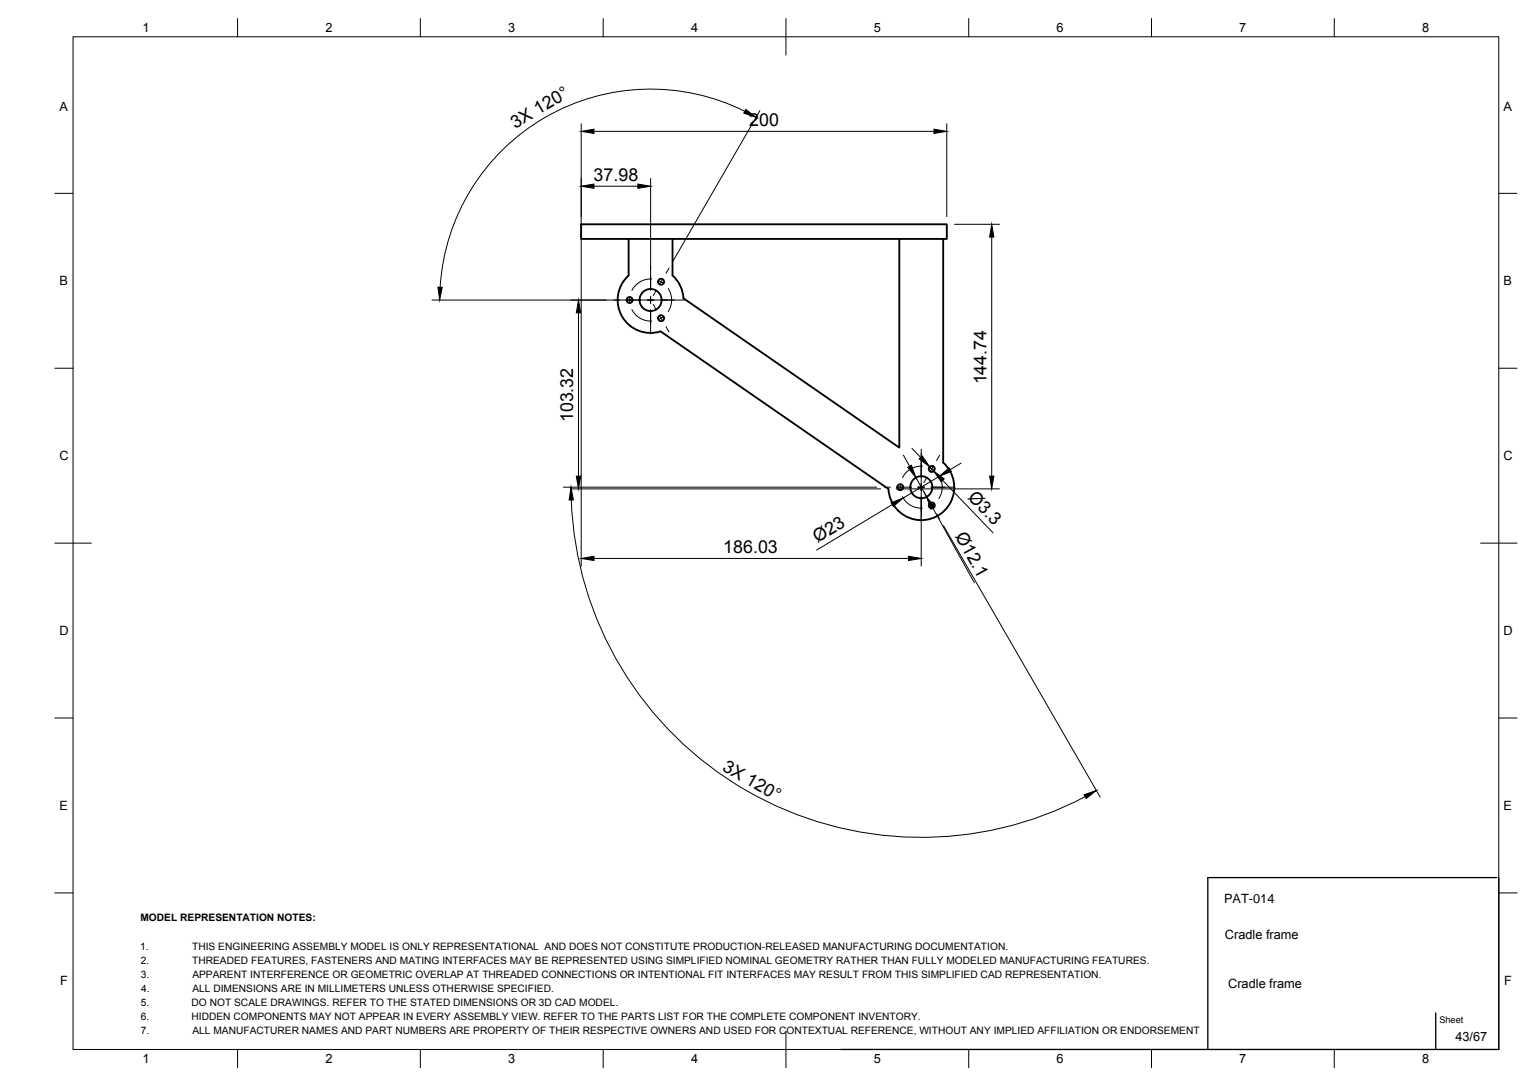
ISO-10303-21;
HEADER;
/* Generated by software containing ST-Developer
 * from STEP Tools, Inc. (www.steptools.com) 
 */

FILE_DESCRIPTION(
/* description */ ('Bin tilter linkage'),
/* implementation_level */ '2;1');

FILE_NAME(
/* name */ 'Cradle frame.step',
/* time_stamp */ '2026-10-28T03:26:24-07:00',
/* author */ (''),
/* organization */ (''),
/* preprocessor_version */ 'ST-DEVELOPER v20.2',
/* originating_system */ 'Autodesk Translation Framework v15.17.0.0',
/* authorisation */ '');

FILE_SCHEMA (('AUTOMOTIVE_DESIGN { 1 0 10303 214 3 1 1 }'));
ENDSEC;

DATA;
#10=MECHANICAL_DESIGN_GEOMETRIC_PRESENTATION_REPRESENTATION('',(#946,#947),#23728);
#727=SHAPE_REPRESENTATION_RELATIONSHIP('SRR','None',#24195,#833);
#833=ADVANCED_BREP_SHAPE_REPRESENTATION('',(#1059,#1060),#23695);
#946=STYLED_ITEM('',(#24744),#1059);
#947=STYLED_ITEM('',(#24744),#1060);
#1059=MANIFOLD_SOLID_BREP('Body1',#12477);
#1060=MANIFOLD_SOLID_BREP('Body2',#12478);
#1395=FACE_BOUND('',#3542,.T.);
#1396=FACE_BOUND('',#3543,.T.);
#1397=FACE_BOUND('',#3544,.T.);
#1398=FACE_BOUND('',#3545,.T.);
#1399=FACE_BOUND('',#3546,.T.);
#1400=FACE_BOUND('',#3547,.T.);
#1401=FACE_BOUND('',#3548,.T.);
#1402=FACE_BOUND('',#3549,.T.);
#1403=FACE_BOUND('',#3557,.T.);
#1404=FACE_BOUND('',#3558,.T.);
#1405=FACE_BOUND('',#3559,.T.);
#1406=FACE_BOUND('',#3560,.T.);
#1407=FACE_BOUND('',#3561,.T.);
#1408=FACE_BOUND('',#3562,.T.);
#1409=FACE_BOUND('',#3563,.T.);
#1410=FACE_BOUND('',#3564,.T.);
#1753=PLANE('',#14973);
#1754=PLANE('',#14974);
#1755=PLANE('',#14975);
#1756=PLANE('',#14982);
#1757=PLANE('',#14984);
#1758=PLANE('',#14985);
#1759=PLANE('',#14986);
#1760=PLANE('',#14987);
#1761=PLANE('',#14990);
#1762=PLANE('',#14991);
#1763=PLANE('',#14992);
#1764=PLANE('',#14993);
#1765=PLANE('',#14994);
#1766=PLANE('',#14995);
#1767=PLANE('',#14996);
#1768=PLANE('',#14997);
#2443=FACE_OUTER_BOUND('',#3528,.T.);
#2444=FACE_OUTER_BOUND('',#3529,.T.);
#2445=FACE_OUTER_BOUND('',#3530,.T.);
#2446=FACE_OUTER_BOUND('',#3531,.T.);
#2447=FACE_OUTER_BOUND('',#3532,.T.);
#2448=FACE_OUTER_BOUND('',#3533,.T.);
#2449=FACE_OUTER_BOUND('',#3534,.T.);
#2450=FACE_OUTER_BOUND('',#3535,.T.);
#2451=FACE_OUTER_BOUND('',#3536,.T.);
#2452=FACE_OUTER_BOUND('',#3537,.T.);
#2453=FACE_OUTER_BOUND('',#3538,.T.);
#2454=FACE_OUTER_BOUND('',#3539,.T.);
#2455=FACE_OUTER_BOUND('',#3540,.T.);
#2456=FACE_OUTER_BOUND('',#3541,.T.);
#2457=FACE_OUTER_BOUND('',#3550,.T.);
#2458=FACE_OUTER_BOUND('',#3551,.T.);
#2459=FACE_OUTER_BOUND('',#3552,.T.);
#2460=FACE_OUTER_BOUND('',#3553,.T.);
#2461=FACE_OUTER_BOUND('',#3554,.T.);
#2462=FACE_OUTER_BOUND('',#3555,.T.);
#2463=FACE_OUTER_BOUND('',#3556,.T.);
#2464=FACE_OUTER_BOUND('',#3565,.T.);
#2465=FACE_OUTER_BOUND('',#3566,.T.);
#2466=FACE_OUTER_BOUND('',#3567,.T.);
#2467=FACE_OUTER_BOUND('',#3568,.T.);
#2468=FACE_OUTER_BOUND('',#3569,.T.);
#2469=FACE_OUTER_BOUND('',#3570,.T.);
#3528=EDGE_LOOP('',(#10411,#10412,#10413,#10414));
#3529=EDGE_LOOP('',(#10415,#10416,#10417,#10418));
#3530=EDGE_LOOP('',(#10419,#10420,#10421,#10422));
#3531=EDGE_LOOP('',(#10423,#10424,#10425,#10426));
#3532=EDGE_LOOP('',(#10427,#10428,#10429,#10430));
#3533=EDGE_LOOP('',(#10431,#10432,#10433,#10434));
#3534=EDGE_LOOP('',(#10435,#10436,#10437,#10438));
#3535=EDGE_LOOP('',(#10439,#10440,#10441,#10442));
#3536=EDGE_LOOP('',(#10443,#10444,#10445,#10446));
#3537=EDGE_LOOP('',(#10447,#10448,#10449,#10450));
#3538=EDGE_LOOP('',(#10451,#10452,#10453,#10454));
#3539=EDGE_LOOP('',(#10455,#10456,#10457,#10458));
#3540=EDGE_LOOP('',(#10459,#10460,#10461,#10462));
#3541=EDGE_LOOP('',(#10463,#10464,#10465,#10466,#10467,#10468,#10469,#10470,
#10471,#10472,#10473));
#3542=EDGE_LOOP('',(#10474));
#3543=EDGE_LOOP('',(#10475));
#3544=EDGE_LOOP('',(#10476));
#3545=EDGE_LOOP('',(#10477));
#3546=EDGE_LOOP('',(#10478));
#3547=EDGE_LOOP('',(#10479));
#3548=EDGE_LOOP('',(#10480));
#3549=EDGE_LOOP('',(#10481));
#3550=EDGE_LOOP('',(#10482,#10483,#10484,#10485));
#3551=EDGE_LOOP('',(#10486,#10487,#10488,#10489));
#3552=EDGE_LOOP('',(#10490,#10491,#10492,#10493));
#3553=EDGE_LOOP('',(#10494,#10495,#10496,#10497));
#3554=EDGE_LOOP('',(#10498,#10499,#10500,#10501));
#3555=EDGE_LOOP('',(#10502,#10503,#10504,#10505));
#3556=EDGE_LOOP('',(#10506,#10507,#10508,#10509,#10510,#10511,#10512,#10513,
#10514,#10515,#10516));
#3557=EDGE_LOOP('',(#10517));
#3558=EDGE_LOOP('',(#10518));
#3559=EDGE_LOOP('',(#10519));
#3560=EDGE_LOOP('',(#10520));
#3561=EDGE_LOOP('',(#10521));
#3562=EDGE_LOOP('',(#10522));
#3563=EDGE_LOOP('',(#10523));
#3564=EDGE_LOOP('',(#10524));
#3565=EDGE_LOOP('',(#10525,#10526,#10527,#10528));
#3566=EDGE_LOOP('',(#10529,#10530,#10531,#10532));
#3567=EDGE_LOOP('',(#10533,#10534,#10535,#10536));
#3568=EDGE_LOOP('',(#10537,#10538,#10539,#10540));
#3569=EDGE_LOOP('',(#10541,#10542,#10543,#10544));
#3570=EDGE_LOOP('',(#10545,#10546,#10547,#10548));
#4269=LINE('',#22436,#4944);
#4270=LINE('',#22442,#4945);
#4271=LINE('',#22448,#4946);
#4272=LINE('',#22454,#4947);
#4273=LINE('',#22460,#4948);
#4274=LINE('',#22466,#4949);
#4275=LINE('',#22472,#4950);
#4276=LINE('',#22478,#4951);
#4277=LINE('',#22483,#4952);
#4278=LINE('',#22485,#4953);
#4279=LINE('',#22487,#4954);
#4280=LINE('',#22488,#4955);
#4281=LINE('',#22492,#4956);
#4282=LINE('',#22494,#4957);
#4283=LINE('',#22496,#4958);
#4284=LINE('',#22497,#4959);
#4285=LINE('',#22499,#4960);
#4286=LINE('',#22500,#4961);
#4287=LINE('',#22505,#4962);
#4288=LINE('',#22511,#4963);
#4289=LINE('',#22515,#4964);
#4290=LINE('',#22517,#4965);
#4291=LINE('',#22519,#4966);
#4292=LINE('',#22521,#4967);
#4293=LINE('',#22524,#4968);
#4294=LINE('',#22527,#4969);
#4295=LINE('',#22529,#4970);
#4296=LINE('',#22530,#4971);
#4297=LINE('',#22533,#4972);
#4298=LINE('',#22535,#4973);
#4299=LINE('',#22536,#4974);
#4300=LINE('',#22538,#4975);
#4301=LINE('',#22540,#4976);
#4302=LINE('',#22544,#4977);
#4303=LINE('',#22546,#4978);
#4304=LINE('',#22551,#4979);
#4305=LINE('',#22553,#4980);
#4306=LINE('',#22555,#4981);
#4307=LINE('',#22556,#4982);
#4308=LINE('',#22559,#4983);
#4309=LINE('',#22561,#4984);
#4310=LINE('',#22562,#4985);
#4311=LINE('',#22565,#4986);
#4312=LINE('',#22567,#4987);
#4313=LINE('',#22568,#4988);
#4314=LINE('',#22570,#4989);
#4315=LINE('',#22571,#4990);
#4944=VECTOR('',#18444,0.164999999999999);
#4945=VECTOR('',#18451,0.164999999999999);
#4946=VECTOR('',#18458,0.164999999999999);
#4947=VECTOR('',#18465,0.605);
#4948=VECTOR('',#18472,0.164999999999999);
#4949=VECTOR('',#18479,0.164999999999999);
#4950=VECTOR('',#18486,0.164999999999999);
#4951=VECTOR('',#18493,0.605);
#4952=VECTOR('',#18498,1.);
#4953=VECTOR('',#18499,1.);
#4954=VECTOR('',#18500,1.);
#4955=VECTOR('',#18501,1.);
#4956=VECTOR('',#18504,1.);
#4957=VECTOR('',#18505,1.);
#4958=VECTOR('',#18506,1.);
#4959=VECTOR('',#18507,1.);
#4960=VECTOR('',#18510,1.);
#4961=VECTOR('',#18511,1.);
#4962=VECTOR('',#18516,1.);
#4963=VECTOR('',#18523,1.);
#4964=VECTOR('',#18528,1.);
#4965=VECTOR('',#18529,1.);
#4966=VECTOR('',#18530,1.);
#4967=VECTOR('',#18531,1.);
#4968=VECTOR('',#18534,1.);
#4969=VECTOR('',#18537,1.);
#4970=VECTOR('',#18538,1.);
#4971=VECTOR('',#18539,1.);
#4972=VECTOR('',#18542,1.);
#4973=VECTOR('',#18543,1.);
#4974=VECTOR('',#18544,1.);
#4975=VECTOR('',#18547,1.);
#4976=VECTOR('',#18550,1.);
#4977=VECTOR('',#18555,1.);
#4978=VECTOR('',#18558,1.);
#4979=VECTOR('',#18563,1.);
#4980=VECTOR('',#18564,1.);
#4981=VECTOR('',#18565,1.);
#4982=VECTOR('',#18566,1.);
#4983=VECTOR('',#18569,1.);
#4984=VECTOR('',#18570,1.);
#4985=VECTOR('',#18571,1.);
#4986=VECTOR('',#18574,1.);
#4987=VECTOR('',#18575,1.);
#4988=VECTOR('',#18576,1.);
#4989=VECTOR('',#18579,1.);
#4990=VECTOR('',#18580,1.);
#5784=CIRCLE('',#14950,0.164999999999999);
#5785=CIRCLE('',#14951,0.164999999999999);
#5786=CIRCLE('',#14953,0.164999999999999);
#5787=CIRCLE('',#14954,0.164999999999999);
#5788=CIRCLE('',#14956,0.164999999999999);
#5789=CIRCLE('',#14957,0.164999999999999);
#5790=CIRCLE('',#14959,0.605);
#5791=CIRCLE('',#14960,0.605);
#5792=CIRCLE('',#14962,0.164999999999999);
#5793=CIRCLE('',#14963,0.164999999999999);
#5794=CIRCLE('',#14965,0.164999999999999);
#5795=CIRCLE('',#14966,0.164999999999999);
#5796=CIRCLE('',#14968,0.164999999999999);
#5797=CIRCLE('',#14969,0.164999999999999);
#5798=CIRCLE('',#14971,0.605);
#5799=CIRCLE('',#14972,0.605);
#5800=CIRCLE('',#14977,1.8);
#5801=CIRCLE('',#14978,1.8);
#5802=CIRCLE('',#14980,1.8);
#5803=CIRCLE('',#14981,1.8);
#5804=CIRCLE('',#14983,1.8);
#5805=CIRCLE('',#14989,1.8);
#6643=VERTEX_POINT('',#22433);
#6644=VERTEX_POINT('',#22435);
#6645=VERTEX_POINT('',#22439);
#6646=VERTEX_POINT('',#22441);
#6647=VERTEX_POINT('',#22445);
#6648=VERTEX_POINT('',#22447);
#6649=VERTEX_POINT('',#22451);
#6650=VERTEX_POINT('',#22453);
#6651=VERTEX_POINT('',#22457);
#6652=VERTEX_POINT('',#22459);
#6653=VERTEX_POINT('',#22463);
#6654=VERTEX_POINT('',#22465);
#6655=VERTEX_POINT('',#22469);
#6656=VERTEX_POINT('',#22471);
#6657=VERTEX_POINT('',#22475);
#6658=VERTEX_POINT('',#22477);
#6659=VERTEX_POINT('',#22481);
#6660=VERTEX_POINT('',#22482);
#6661=VERTEX_POINT('',#22484);
#6662=VERTEX_POINT('',#22486);
#6663=VERTEX_POINT('',#22490);
#6664=VERTEX_POINT('',#22491);
#6665=VERTEX_POINT('',#22493);
#6666=VERTEX_POINT('',#22495);
#6667=VERTEX_POINT('',#22502);
#6668=VERTEX_POINT('',#22504);
#6669=VERTEX_POINT('',#22508);
#6670=VERTEX_POINT('',#22510);
#6671=VERTEX_POINT('',#22514);
#6672=VERTEX_POINT('',#22516);
#6673=VERTEX_POINT('',#22518);
#6674=VERTEX_POINT('',#22520);
#6675=VERTEX_POINT('',#22522);
#6676=VERTEX_POINT('',#22526);
#6677=VERTEX_POINT('',#22528);
#6678=VERTEX_POINT('',#22532);
#6679=VERTEX_POINT('',#22534);
#6680=VERTEX_POINT('',#22542);
#6681=VERTEX_POINT('',#22549);
#6682=VERTEX_POINT('',#22550);
#6683=VERTEX_POINT('',#22552);
#6684=VERTEX_POINT('',#22554);
#6685=VERTEX_POINT('',#22558);
#6686=VERTEX_POINT('',#22560);
#6687=VERTEX_POINT('',#22564);
#6688=VERTEX_POINT('',#22566);
#7945=EDGE_CURVE('',#6643,#6643,#5784,.T.);
#7946=EDGE_CURVE('',#6643,#6644,#4269,.T.);
#7947=EDGE_CURVE('',#6644,#6644,#5785,.T.);
#7948=EDGE_CURVE('',#6645,#6645,#5786,.T.);
#7949=EDGE_CURVE('',#6645,#6646,#4270,.T.);
#7950=EDGE_CURVE('',#6646,#6646,#5787,.T.);
#7951=EDGE_CURVE('',#6647,#6647,#5788,.T.);
#7952=EDGE_CURVE('',#6647,#6648,#4271,.T.);
#7953=EDGE_CURVE('',#6648,#6648,#5789,.T.);
#7954=EDGE_CURVE('',#6649,#6649,#5790,.T.);
#7955=EDGE_CURVE('',#6649,#6650,#4272,.T.);
#7956=EDGE_CURVE('',#6650,#6650,#5791,.T.);
#7957=EDGE_CURVE('',#6651,#6651,#5792,.T.);
#7958=EDGE_CURVE('',#6651,#6652,#4273,.T.);
#7959=EDGE_CURVE('',#6652,#6652,#5793,.T.);
#7960=EDGE_CURVE('',#6653,#6653,#5794,.T.);
#7961=EDGE_CURVE('',#6653,#6654,#4274,.T.);
#7962=EDGE_CURVE('',#6654,#6654,#5795,.T.);
#7963=EDGE_CURVE('',#6655,#6655,#5796,.T.);
#7964=EDGE_CURVE('',#6655,#6656,#4275,.T.);
#7965=EDGE_CURVE('',#6656,#6656,#5797,.T.);
#7966=EDGE_CURVE('',#6657,#6657,#5798,.T.);
#7967=EDGE_CURVE('',#6657,#6658,#4276,.T.);
#7968=EDGE_CURVE('',#6658,#6658,#5799,.T.);
#7969=EDGE_CURVE('',#6659,#6660,#4277,.T.);
#7970=EDGE_CURVE('',#6661,#6659,#4278,.T.);
#7971=EDGE_CURVE('',#6661,#6662,#4279,.T.);
#7972=EDGE_CURVE('',#6660,#6662,#4280,.T.);
#7973=EDGE_CURVE('',#6663,#6664,#4281,.T.);
#7974=EDGE_CURVE('',#6665,#6663,#4282,.T.);
#7975=EDGE_CURVE('',#6666,#6665,#4283,.T.);
#7976=EDGE_CURVE('',#6664,#6666,#4284,.T.);
#7977=EDGE_CURVE('',#6666,#6661,#4285,.T.);
#7978=EDGE_CURVE('',#6662,#6665,#4286,.T.);
#7979=EDGE_CURVE('',#6667,#6660,#5800,.T.);
#7980=EDGE_CURVE('',#6668,#6667,#4287,.T.);
#7981=EDGE_CURVE('',#6668,#6659,#5801,.T.);
#7982=EDGE_CURVE('',#6664,#6669,#5802,.T.);
#7983=EDGE_CURVE('',#6670,#6669,#4288,.T.);
#7984=EDGE_CURVE('',#6663,#6670,#5803,.T.);
#7985=EDGE_CURVE('',#6671,#6668,#4289,.T.);
#7986=EDGE_CURVE('',#6671,#6672,#4290,.T.);
#7987=EDGE_CURVE('',#6672,#6673,#4291,.T.);
#7988=EDGE_CURVE('',#6673,#6674,#4292,.T.);
#7989=EDGE_CURVE('',#6675,#6674,#5804,.T.);
#7990=EDGE_CURVE('',#6669,#6675,#4293,.T.);
#7991=EDGE_CURVE('',#6674,#6676,#4294,.T.);
#7992=EDGE_CURVE('',#6673,#6677,#4295,.T.);
#7993=EDGE_CURVE('',#6676,#6677,#4296,.T.);
#7994=EDGE_CURVE('',#6678,#6671,#4297,.T.);
#7995=EDGE_CURVE('',#6679,#6678,#4298,.T.);
#7996=EDGE_CURVE('',#6672,#6679,#4299,.T.);
#7997=EDGE_CURVE('',#6677,#6679,#4300,.T.);
#7998=EDGE_CURVE('',#6678,#6667,#4301,.T.);
#7999=EDGE_CURVE('',#6680,#6676,#5805,.T.);
#8000=EDGE_CURVE('',#6675,#6680,#4302,.T.);
#8001=EDGE_CURVE('',#6670,#6680,#4303,.T.);
#8002=EDGE_CURVE('',#6681,#6682,#4304,.T.);
#8003=EDGE_CURVE('',#6682,#6683,#4305,.T.);
#8004=EDGE_CURVE('',#6684,#6683,#4306,.T.);
#8005=EDGE_CURVE('',#6681,#6684,#4307,.T.);
#8006=EDGE_CURVE('',#6685,#6681,#4308,.T.);
#8007=EDGE_CURVE('',#6686,#6684,#4309,.T.);
#8008=EDGE_CURVE('',#6685,#6686,#4310,.T.);
#8009=EDGE_CURVE('',#6687,#6685,#4311,.T.);
#8010=EDGE_CURVE('',#6688,#6686,#4312,.T.);
#8011=EDGE_CURVE('',#6687,#6688,#4313,.T.);
#8012=EDGE_CURVE('',#6682,#6687,#4314,.T.);
#8013=EDGE_CURVE('',#6683,#6688,#4315,.T.);
#10411=ORIENTED_EDGE('',*,*,#7945,.F.);
#10412=ORIENTED_EDGE('',*,*,#7946,.T.);
#10413=ORIENTED_EDGE('',*,*,#7947,.F.);
#10414=ORIENTED_EDGE('',*,*,#7946,.F.);
#10415=ORIENTED_EDGE('',*,*,#7948,.F.);
#10416=ORIENTED_EDGE('',*,*,#7949,.T.);
#10417=ORIENTED_EDGE('',*,*,#7950,.F.);
#10418=ORIENTED_EDGE('',*,*,#7949,.F.);
#10419=ORIENTED_EDGE('',*,*,#7951,.F.);
#10420=ORIENTED_EDGE('',*,*,#7952,.T.);
#10421=ORIENTED_EDGE('',*,*,#7953,.F.);
#10422=ORIENTED_EDGE('',*,*,#7952,.F.);
#10423=ORIENTED_EDGE('',*,*,#7954,.F.);
#10424=ORIENTED_EDGE('',*,*,#7955,.T.);
#10425=ORIENTED_EDGE('',*,*,#7956,.F.);
#10426=ORIENTED_EDGE('',*,*,#7955,.F.);
#10427=ORIENTED_EDGE('',*,*,#7957,.F.);
#10428=ORIENTED_EDGE('',*,*,#7958,.T.);
#10429=ORIENTED_EDGE('',*,*,#7959,.F.);
#10430=ORIENTED_EDGE('',*,*,#7958,.F.);
#10431=ORIENTED_EDGE('',*,*,#7960,.F.);
#10432=ORIENTED_EDGE('',*,*,#7961,.T.);
#10433=ORIENTED_EDGE('',*,*,#7962,.F.);
#10434=ORIENTED_EDGE('',*,*,#7961,.F.);
#10435=ORIENTED_EDGE('',*,*,#7963,.F.);
#10436=ORIENTED_EDGE('',*,*,#7964,.T.);
#10437=ORIENTED_EDGE('',*,*,#7965,.F.);
#10438=ORIENTED_EDGE('',*,*,#7964,.F.);
#10439=ORIENTED_EDGE('',*,*,#7966,.F.);
#10440=ORIENTED_EDGE('',*,*,#7967,.T.);
#10441=ORIENTED_EDGE('',*,*,#7968,.F.);
#10442=ORIENTED_EDGE('',*,*,#7967,.F.);
#10443=ORIENTED_EDGE('',*,*,#7969,.F.);
#10444=ORIENTED_EDGE('',*,*,#7970,.F.);
#10445=ORIENTED_EDGE('',*,*,#7971,.T.);
#10446=ORIENTED_EDGE('',*,*,#7972,.F.);
#10447=ORIENTED_EDGE('',*,*,#7973,.F.);
#10448=ORIENTED_EDGE('',*,*,#7974,.F.);
#10449=ORIENTED_EDGE('',*,*,#7975,.F.);
#10450=ORIENTED_EDGE('',*,*,#7976,.F.);
#10451=ORIENTED_EDGE('',*,*,#7977,.F.);
#10452=ORIENTED_EDGE('',*,*,#7975,.T.);
#10453=ORIENTED_EDGE('',*,*,#7978,.F.);
#10454=ORIENTED_EDGE('',*,*,#7971,.F.);
#10455=ORIENTED_EDGE('',*,*,#7969,.T.);
#10456=ORIENTED_EDGE('',*,*,#7979,.F.);
#10457=ORIENTED_EDGE('',*,*,#7980,.F.);
#10458=ORIENTED_EDGE('',*,*,#7981,.T.);
#10459=ORIENTED_EDGE('',*,*,#7973,.T.);
#10460=ORIENTED_EDGE('',*,*,#7982,.T.);
#10461=ORIENTED_EDGE('',*,*,#7983,.F.);
#10462=ORIENTED_EDGE('',*,*,#7984,.F.);
#10463=ORIENTED_EDGE('',*,*,#7981,.F.);
#10464=ORIENTED_EDGE('',*,*,#7985,.F.);
#10465=ORIENTED_EDGE('',*,*,#7986,.T.);
#10466=ORIENTED_EDGE('',*,*,#7987,.T.);
#10467=ORIENTED_EDGE('',*,*,#7988,.T.);
#10468=ORIENTED_EDGE('',*,*,#7989,.F.);
#10469=ORIENTED_EDGE('',*,*,#7990,.F.);
#10470=ORIENTED_EDGE('',*,*,#7982,.F.);
#10471=ORIENTED_EDGE('',*,*,#7976,.T.);
#10472=ORIENTED_EDGE('',*,*,#7977,.T.);
#10473=ORIENTED_EDGE('',*,*,#7970,.T.);
#10474=ORIENTED_EDGE('',*,*,#7966,.T.);
#10475=ORIENTED_EDGE('',*,*,#7963,.T.);
#10476=ORIENTED_EDGE('',*,*,#7960,.T.);
#10477=ORIENTED_EDGE('',*,*,#7957,.T.);
#10478=ORIENTED_EDGE('',*,*,#7954,.T.);
#10479=ORIENTED_EDGE('',*,*,#7951,.T.);
#10480=ORIENTED_EDGE('',*,*,#7948,.T.);
#10481=ORIENTED_EDGE('',*,*,#7945,.T.);
#10482=ORIENTED_EDGE('',*,*,#7991,.F.);
#10483=ORIENTED_EDGE('',*,*,#7988,.F.);
#10484=ORIENTED_EDGE('',*,*,#7992,.T.);
#10485=ORIENTED_EDGE('',*,*,#7993,.F.);
#10486=ORIENTED_EDGE('',*,*,#7994,.F.);
#10487=ORIENTED_EDGE('',*,*,#7995,.F.);
#10488=ORIENTED_EDGE('',*,*,#7996,.F.);
#10489=ORIENTED_EDGE('',*,*,#7986,.F.);
#10490=ORIENTED_EDGE('',*,*,#7987,.F.);
#10491=ORIENTED_EDGE('',*,*,#7996,.T.);
#10492=ORIENTED_EDGE('',*,*,#7997,.F.);
#10493=ORIENTED_EDGE('',*,*,#7992,.F.);
#10494=ORIENTED_EDGE('',*,*,#7994,.T.);
#10495=ORIENTED_EDGE('',*,*,#7985,.T.);
#10496=ORIENTED_EDGE('',*,*,#7980,.T.);
#10497=ORIENTED_EDGE('',*,*,#7998,.F.);
#10498=ORIENTED_EDGE('',*,*,#7991,.T.);
#10499=ORIENTED_EDGE('',*,*,#7999,.F.);
#10500=ORIENTED_EDGE('',*,*,#8000,.F.);
#10501=ORIENTED_EDGE('',*,*,#7989,.T.);
#10502=ORIENTED_EDGE('',*,*,#7983,.T.);
#10503=ORIENTED_EDGE('',*,*,#7990,.T.);
#10504=ORIENTED_EDGE('',*,*,#8000,.T.);
#10505=ORIENTED_EDGE('',*,*,#8001,.F.);
#10506=ORIENTED_EDGE('',*,*,#7984,.T.);
#10507=ORIENTED_EDGE('',*,*,#8001,.T.);
#10508=ORIENTED_EDGE('',*,*,#7999,.T.);
#10509=ORIENTED_EDGE('',*,*,#7993,.T.);
#10510=ORIENTED_EDGE('',*,*,#7997,.T.);
#10511=ORIENTED_EDGE('',*,*,#7995,.T.);
#10512=ORIENTED_EDGE('',*,*,#7998,.T.);
#10513=ORIENTED_EDGE('',*,*,#7979,.T.);
#10514=ORIENTED_EDGE('',*,*,#7972,.T.);
#10515=ORIENTED_EDGE('',*,*,#7978,.T.);
#10516=ORIENTED_EDGE('',*,*,#7974,.T.);
#10517=ORIENTED_EDGE('',*,*,#7968,.T.);
#10518=ORIENTED_EDGE('',*,*,#7965,.T.);
#10519=ORIENTED_EDGE('',*,*,#7962,.T.);
#10520=ORIENTED_EDGE('',*,*,#7959,.T.);
#10521=ORIENTED_EDGE('',*,*,#7956,.T.);
#10522=ORIENTED_EDGE('',*,*,#7953,.T.);
#10523=ORIENTED_EDGE('',*,*,#7950,.T.);
#10524=ORIENTED_EDGE('',*,*,#7947,.T.);
#10525=ORIENTED_EDGE('',*,*,#8002,.T.);
#10526=ORIENTED_EDGE('',*,*,#8003,.T.);
#10527=ORIENTED_EDGE('',*,*,#8004,.F.);
#10528=ORIENTED_EDGE('',*,*,#8005,.F.);
#10529=ORIENTED_EDGE('',*,*,#8006,.T.);
#10530=ORIENTED_EDGE('',*,*,#8005,.T.);
#10531=ORIENTED_EDGE('',*,*,#8007,.F.);
#10532=ORIENTED_EDGE('',*,*,#8008,.F.);
#10533=ORIENTED_EDGE('',*,*,#8009,.T.);
#10534=ORIENTED_EDGE('',*,*,#8008,.T.);
#10535=ORIENTED_EDGE('',*,*,#8010,.F.);
#10536=ORIENTED_EDGE('',*,*,#8011,.F.);
#10537=ORIENTED_EDGE('',*,*,#8012,.T.);
#10538=ORIENTED_EDGE('',*,*,#8011,.T.);
#10539=ORIENTED_EDGE('',*,*,#8013,.F.);
#10540=ORIENTED_EDGE('',*,*,#8003,.F.);
#10541=ORIENTED_EDGE('',*,*,#8013,.T.);
#10542=ORIENTED_EDGE('',*,*,#8010,.T.);
#10543=ORIENTED_EDGE('',*,*,#8007,.T.);
#10544=ORIENTED_EDGE('',*,*,#8004,.T.);
#10545=ORIENTED_EDGE('',*,*,#8012,.F.);
#10546=ORIENTED_EDGE('',*,*,#8002,.F.);
#10547=ORIENTED_EDGE('',*,*,#8006,.F.);
#10548=ORIENTED_EDGE('',*,*,#8009,.F.);
#11535=CYLINDRICAL_SURFACE('',#14949,0.164999999999999);
#11536=CYLINDRICAL_SURFACE('',#14952,0.164999999999999);
#11537=CYLINDRICAL_SURFACE('',#14955,0.164999999999999);
#11538=CYLINDRICAL_SURFACE('',#14958,0.605);
#11539=CYLINDRICAL_SURFACE('',#14961,0.164999999999999);
#11540=CYLINDRICAL_SURFACE('',#14964,0.164999999999999);
#11541=CYLINDRICAL_SURFACE('',#14967,0.164999999999999);
#11542=CYLINDRICAL_SURFACE('',#14970,0.605);
#11543=CYLINDRICAL_SURFACE('',#14976,1.8);
#11544=CYLINDRICAL_SURFACE('',#14979,1.8);
#11545=CYLINDRICAL_SURFACE('',#14988,1.8);
#12168=ADVANCED_FACE('',(#2443),#11535,.F.);
#12169=ADVANCED_FACE('',(#2444),#11536,.F.);
#12170=ADVANCED_FACE('',(#2445),#11537,.F.);
#12171=ADVANCED_FACE('',(#2446),#11538,.F.);
#12172=ADVANCED_FACE('',(#2447),#11539,.F.);
#12173=ADVANCED_FACE('',(#2448),#11540,.F.);
#12174=ADVANCED_FACE('',(#2449),#11541,.F.);
#12175=ADVANCED_FACE('',(#2450),#11542,.F.);
#12176=ADVANCED_FACE('',(#2451),#1753,.T.);
#12177=ADVANCED_FACE('',(#2452),#1754,.T.);
#12178=ADVANCED_FACE('',(#2453),#1755,.T.);
#12179=ADVANCED_FACE('',(#2454),#11543,.T.);
#12180=ADVANCED_FACE('',(#2455),#11544,.T.);
#12181=ADVANCED_FACE('',(#2456,#1395,#1396,#1397,#1398,#1399,#1400,#1401,
#1402),#1756,.F.);
#12182=ADVANCED_FACE('',(#2457),#1757,.T.);
#12183=ADVANCED_FACE('',(#2458),#1758,.T.);
#12184=ADVANCED_FACE('',(#2459),#1759,.T.);
#12185=ADVANCED_FACE('',(#2460),#1760,.T.);
#12186=ADVANCED_FACE('',(#2461),#11545,.T.);
#12187=ADVANCED_FACE('',(#2462),#1761,.T.);
#12188=ADVANCED_FACE('',(#2463,#1403,#1404,#1405,#1406,#1407,#1408,#1409,
#1410),#1762,.T.);
#12189=ADVANCED_FACE('',(#2464),#1763,.T.);
#12190=ADVANCED_FACE('',(#2465),#1764,.T.);
#12191=ADVANCED_FACE('',(#2466),#1765,.T.);
#12192=ADVANCED_FACE('',(#2467),#1766,.T.);
#12193=ADVANCED_FACE('',(#2468),#1767,.T.);
#12194=ADVANCED_FACE('',(#2469),#1768,.F.);
#12477=CLOSED_SHELL('',(#12168,#12169,#12170,#12171,#12172,#12173,#12174,
#12175,#12176,#12177,#12178,#12179,#12180,#12181,#12182,#12183,#12184,#12185,
#12186,#12187,#12188));
#12478=CLOSED_SHELL('',(#12189,#12190,#12191,#12192,#12193,#12194));
#14948=AXIS2_PLACEMENT_3D('',#22431,#18438,#18439);
#14949=AXIS2_PLACEMENT_3D('',#22432,#18440,#18441);
#14950=AXIS2_PLACEMENT_3D('',#22434,#18442,#18443);
#14951=AXIS2_PLACEMENT_3D('',#22437,#18445,#18446);
#14952=AXIS2_PLACEMENT_3D('',#22438,#18447,#18448);
#14953=AXIS2_PLACEMENT_3D('',#22440,#18449,#18450);
#14954=AXIS2_PLACEMENT_3D('',#22443,#18452,#18453);
#14955=AXIS2_PLACEMENT_3D('',#22444,#18454,#18455);
#14956=AXIS2_PLACEMENT_3D('',#22446,#18456,#18457);
#14957=AXIS2_PLACEMENT_3D('',#22449,#18459,#18460);
#14958=AXIS2_PLACEMENT_3D('',#22450,#18461,#18462);
#14959=AXIS2_PLACEMENT_3D('',#22452,#18463,#18464);
#14960=AXIS2_PLACEMENT_3D('',#22455,#18466,#18467);
#14961=AXIS2_PLACEMENT_3D('',#22456,#18468,#18469);
#14962=AXIS2_PLACEMENT_3D('',#22458,#18470,#18471);
#14963=AXIS2_PLACEMENT_3D('',#22461,#18473,#18474);
#14964=AXIS2_PLACEMENT_3D('',#22462,#18475,#18476);
#14965=AXIS2_PLACEMENT_3D('',#22464,#18477,#18478);
#14966=AXIS2_PLACEMENT_3D('',#22467,#18480,#18481);
#14967=AXIS2_PLACEMENT_3D('',#22468,#18482,#18483);
#14968=AXIS2_PLACEMENT_3D('',#22470,#18484,#18485);
#14969=AXIS2_PLACEMENT_3D('',#22473,#18487,#18488);
#14970=AXIS2_PLACEMENT_3D('',#22474,#18489,#18490);
#14971=AXIS2_PLACEMENT_3D('',#22476,#18491,#18492);
#14972=AXIS2_PLACEMENT_3D('',#22479,#18494,#18495);
#14973=AXIS2_PLACEMENT_3D('',#22480,#18496,#18497);
#14974=AXIS2_PLACEMENT_3D('',#22489,#18502,#18503);
#14975=AXIS2_PLACEMENT_3D('',#22498,#18508,#18509);
#14976=AXIS2_PLACEMENT_3D('',#22501,#18512,#18513);
#14977=AXIS2_PLACEMENT_3D('',#22503,#18514,#18515);
#14978=AXIS2_PLACEMENT_3D('',#22506,#18517,#18518);
#14979=AXIS2_PLACEMENT_3D('',#22507,#18519,#18520);
#14980=AXIS2_PLACEMENT_3D('',#22509,#18521,#18522);
#14981=AXIS2_PLACEMENT_3D('',#22512,#18524,#18525);
#14982=AXIS2_PLACEMENT_3D('',#22513,#18526,#18527);
#14983=AXIS2_PLACEMENT_3D('',#22523,#18532,#18533);
#14984=AXIS2_PLACEMENT_3D('',#22525,#18535,#18536);
#14985=AXIS2_PLACEMENT_3D('',#22531,#18540,#18541);
#14986=AXIS2_PLACEMENT_3D('',#22537,#18545,#18546);
#14987=AXIS2_PLACEMENT_3D('',#22539,#18548,#18549);
#14988=AXIS2_PLACEMENT_3D('',#22541,#18551,#18552);
#14989=AXIS2_PLACEMENT_3D('',#22543,#18553,#18554);
#14990=AXIS2_PLACEMENT_3D('',#22545,#18556,#18557);
#14991=AXIS2_PLACEMENT_3D('',#22547,#18559,#18560);
#14992=AXIS2_PLACEMENT_3D('',#22548,#18561,#18562);
#14993=AXIS2_PLACEMENT_3D('',#22557,#18567,#18568);
#14994=AXIS2_PLACEMENT_3D('',#22563,#18572,#18573);
#14995=AXIS2_PLACEMENT_3D('',#22569,#18577,#18578);
#14996=AXIS2_PLACEMENT_3D('',#22572,#18581,#18582);
#14997=AXIS2_PLACEMENT_3D('',#22573,#18583,#18584);
#18438=DIRECTION('axis',(0.,0.,1.));
#18439=DIRECTION('refdir',(1.,0.,0.));
#18440=DIRECTION('center_axis',(0.,1.,0.));
#18441=DIRECTION('ref_axis',(1.,0.,0.));
#18442=DIRECTION('center_axis',(0.,1.,0.));
#18443=DIRECTION('ref_axis',(1.,0.,0.));
#18444=DIRECTION('',(0.,1.,0.));
#18445=DIRECTION('center_axis',(0.,-1.,0.));
#18446=DIRECTION('ref_axis',(1.,0.,0.));
#18447=DIRECTION('center_axis',(0.,1.,0.));
#18448=DIRECTION('ref_axis',(1.,0.,0.));
#18449=DIRECTION('center_axis',(0.,1.,0.));
#18450=DIRECTION('ref_axis',(1.,0.,0.));
#18451=DIRECTION('',(0.,1.,0.));
#18452=DIRECTION('center_axis',(0.,-1.,0.));
#18453=DIRECTION('ref_axis',(1.,0.,0.));
#18454=DIRECTION('center_axis',(0.,1.,0.));
#18455=DIRECTION('ref_axis',(1.,0.,0.));
#18456=DIRECTION('center_axis',(0.,1.,0.));
#18457=DIRECTION('ref_axis',(1.,0.,0.));
#18458=DIRECTION('',(0.,1.,0.));
#18459=DIRECTION('center_axis',(0.,-1.,0.));
#18460=DIRECTION('ref_axis',(1.,0.,0.));
#18461=DIRECTION('center_axis',(0.,1.,0.));
#18462=DIRECTION('ref_axis',(1.,0.,0.));
#18463=DIRECTION('center_axis',(0.,1.,0.));
#18464=DIRECTION('ref_axis',(1.,0.,0.));
#18465=DIRECTION('',(0.,1.,0.));
#18466=DIRECTION('center_axis',(0.,-1.,0.));
#18467=DIRECTION('ref_axis',(1.,0.,0.));
#18468=DIRECTION('center_axis',(0.,1.,0.));
#18469=DIRECTION('ref_axis',(1.,0.,0.));
#18470=DIRECTION('center_axis',(0.,1.,0.));
#18471=DIRECTION('ref_axis',(1.,0.,0.));
#18472=DIRECTION('',(0.,1.,0.));
#18473=DIRECTION('center_axis',(0.,-1.,0.));
#18474=DIRECTION('ref_axis',(1.,0.,0.));
#18475=DIRECTION('center_axis',(0.,1.,0.));
#18476=DIRECTION('ref_axis',(1.,0.,0.));
#18477=DIRECTION('center_axis',(0.,1.,0.));
#18478=DIRECTION('ref_axis',(1.,0.,0.));
#18479=DIRECTION('',(0.,1.,0.));
#18480=DIRECTION('center_axis',(0.,-1.,0.));
#18481=DIRECTION('ref_axis',(1.,0.,0.));
#18482=DIRECTION('center_axis',(0.,1.,0.));
#18483=DIRECTION('ref_axis',(1.,0.,0.));
#18484=DIRECTION('center_axis',(0.,1.,0.));
#18485=DIRECTION('ref_axis',(1.,0.,0.));
#18486=DIRECTION('',(0.,1.,0.));
#18487=DIRECTION('center_axis',(0.,-1.,0.));
#18488=DIRECTION('ref_axis',(1.,0.,0.));
#18489=DIRECTION('center_axis',(0.,1.,0.));
#18490=DIRECTION('ref_axis',(1.,0.,0.));
#18491=DIRECTION('center_axis',(0.,1.,0.));
#18492=DIRECTION('ref_axis',(1.,0.,0.));
#18493=DIRECTION('',(0.,1.,0.));
#18494=DIRECTION('center_axis',(0.,-1.,0.));
#18495=DIRECTION('ref_axis',(1.,0.,0.));
#18496=DIRECTION('center_axis',(-1.,0.,0.));
#18497=DIRECTION('ref_axis',(0.,0.,1.));
#18498=DIRECTION('',(0.,1.,0.));
#18499=DIRECTION('',(0.,0.,-1.));
#18500=DIRECTION('',(0.,1.,0.));
#18501=DIRECTION('',(0.,0.,1.));
#18502=DIRECTION('center_axis',(1.,0.,0.));
#18503=DIRECTION('ref_axis',(0.,0.,-1.));
#18504=DIRECTION('',(0.,-1.,0.));
#18505=DIRECTION('',(0.,0.,-1.));
#18506=DIRECTION('',(0.,1.,0.));
#18507=DIRECTION('',(0.,0.,1.));
#18508=DIRECTION('center_axis',(0.,0.,1.));
#18509=DIRECTION('ref_axis',(1.,0.,0.));
#18510=DIRECTION('',(-1.,0.,0.));
#18511=DIRECTION('',(1.,0.,0.));
#18512=DIRECTION('center_axis',(0.,1.,0.));
#18513=DIRECTION('ref_axis',(1.,0.,0.));
#18514=DIRECTION('center_axis',(0.,1.,0.));
#18515=DIRECTION('ref_axis',(1.,0.,0.));
#18516=DIRECTION('',(0.,1.,0.));
#18517=DIRECTION('center_axis',(0.,1.,0.));
#18518=DIRECTION('ref_axis',(1.,0.,0.));
#18519=DIRECTION('center_axis',(0.,1.,0.));
#18520=DIRECTION('ref_axis',(1.,0.,0.));
#18521=DIRECTION('center_axis',(0.,1.,0.));
#18522=DIRECTION('ref_axis',(1.,0.,0.));
#18523=DIRECTION('',(0.,-1.,0.));
#18524=DIRECTION('center_axis',(0.,1.,0.));
#18525=DIRECTION('ref_axis',(1.,0.,0.));
#18526=DIRECTION('center_axis',(0.,1.,0.));
#18527=DIRECTION('ref_axis',(1.,0.,0.));
#18528=DIRECTION('',(0.822508459509058,0.,0.568752876068364));
#18529=DIRECTION('',(0.,0.,1.));
#18530=DIRECTION('',(-1.,0.,0.));
#18531=DIRECTION('',(0.,0.,-1.));
#18532=DIRECTION('center_axis',(0.,1.,0.));
#18533=DIRECTION('ref_axis',(1.,0.,0.));
#18534=DIRECTION('',(-0.822508459509058,0.,-0.568752876068364));
#18535=DIRECTION('center_axis',(-1.,0.,0.));
#18536=DIRECTION('ref_axis',(0.,0.,1.));
#18537=DIRECTION('',(0.,1.,0.));
#18538=DIRECTION('',(0.,1.,0.));
#18539=DIRECTION('',(0.,0.,1.));
#18540=DIRECTION('center_axis',(1.,0.,0.));
#18541=DIRECTION('ref_axis',(0.,0.,-1.));
#18542=DIRECTION('',(0.,-1.,0.));
#18543=DIRECTION('',(0.,0.,-1.));
#18544=DIRECTION('',(0.,1.,0.));
#18545=DIRECTION('center_axis',(0.,0.,1.));
#18546=DIRECTION('ref_axis',(1.,0.,0.));
#18547=DIRECTION('',(1.,0.,0.));
#18548=DIRECTION('center_axis',(-0.568752876068364,0.,0.822508459509058));
#18549=DIRECTION('ref_axis',(0.822508459509058,0.,0.568752876068364));
#18550=DIRECTION('',(0.822508459509058,0.,0.568752876068364));
#18551=DIRECTION('center_axis',(0.,1.,0.));
#18552=DIRECTION('ref_axis',(-0.432056364839205,0.,-0.901846604252592));
#18553=DIRECTION('center_axis',(0.,1.,0.));
#18554=DIRECTION('ref_axis',(1.,0.,0.));
#18555=DIRECTION('',(0.,1.,0.));
#18556=DIRECTION('center_axis',(0.568752876068364,0.,-0.822508459509058));
#18557=DIRECTION('ref_axis',(-0.822508459509058,0.,-0.568752876068364));
#18558=DIRECTION('',(-0.822508459509058,0.,-0.568752876068364));
#18559=DIRECTION('center_axis',(0.,1.,0.));
#18560=DIRECTION('ref_axis',(0.,0.,1.));
#18561=DIRECTION('center_axis',(0.,1.,0.));
#18562=DIRECTION('ref_axis',(-1.,0.,0.));
#18563=DIRECTION('',(-1.,0.,0.));
#18564=DIRECTION('',(0.,0.,1.));
#18565=DIRECTION('',(-1.,0.,0.));
#18566=DIRECTION('',(0.,0.,1.));
#18567=DIRECTION('center_axis',(1.,0.,0.));
#18568=DIRECTION('ref_axis',(0.,1.,0.));
#18569=DIRECTION('',(0.,1.,0.));
#18570=DIRECTION('',(0.,1.,0.));
#18571=DIRECTION('',(0.,0.,1.));
#18572=DIRECTION('center_axis',(0.,-1.,0.));
#18573=DIRECTION('ref_axis',(1.,0.,0.));
#18574=DIRECTION('',(1.,0.,0.));
#18575=DIRECTION('',(1.,0.,0.));
#18576=DIRECTION('',(0.,0.,1.));
#18577=DIRECTION('center_axis',(-1.,0.,0.));
#18578=DIRECTION('ref_axis',(0.,-1.,0.));
#18579=DIRECTION('',(0.,-1.,0.));
#18580=DIRECTION('',(0.,-1.,0.));
#18581=DIRECTION('center_axis',(0.,0.,1.));
#18582=DIRECTION('ref_axis',(1.,0.,0.));
#18583=DIRECTION('center_axis',(0.,0.,1.));
#18584=DIRECTION('ref_axis',(1.,0.,0.));
#22431=CARTESIAN_POINT('',(0.,0.,0.));
#22432=CARTESIAN_POINT('Origin',(25.3520784790221,2.4,28.6577532024872));
#22433=CARTESIAN_POINT('',(25.1870784790221,2.5,28.6577532024872));
#22434=CARTESIAN_POINT('Origin',(25.3520784790221,2.5,28.6577532024872));
#22435=CARTESIAN_POINT('',(25.1870784790221,3.5,28.6577532024872));
#22436=CARTESIAN_POINT('',(25.1870784790221,2.4,28.6577532024872));
#22437=CARTESIAN_POINT('Origin',(25.3520784790221,3.5,28.6577532024872));
#22438=CARTESIAN_POINT('Origin',(23.6270784790221,2.4,29.6536824168393));
#22439=CARTESIAN_POINT('',(23.4620784790221,2.5,29.6536824168393));
#22440=CARTESIAN_POINT('Origin',(23.6270784790221,2.5,29.6536824168393));
#22441=CARTESIAN_POINT('',(23.4620784790221,3.5,29.6536824168393));
#22442=CARTESIAN_POINT('',(23.4620784790221,2.4,29.6536824168393));
#22443=CARTESIAN_POINT('Origin',(23.6270784790221,3.5,29.6536824168393));
#22444=CARTESIAN_POINT('Origin',(23.6270784790221,2.4,27.6618239881351));
#22445=CARTESIAN_POINT('',(23.4620784790221,2.5,27.6618239881351));
#22446=CARTESIAN_POINT('Origin',(23.6270784790221,2.5,27.6618239881351));
#22447=CARTESIAN_POINT('',(23.4620784790221,3.5,27.6618239881351));
#22448=CARTESIAN_POINT('',(23.4620784790221,2.4,27.6618239881351));
#22449=CARTESIAN_POINT('Origin',(23.6270784790221,3.5,27.6618239881351));
#22450=CARTESIAN_POINT('Origin',(24.2020784790221,2.4,28.6577532024872));
#22451=CARTESIAN_POINT('',(23.5970784790221,2.5,28.6577532024872));
#22452=CARTESIAN_POINT('Origin',(24.2020784790221,2.5,28.6577532024872));
#22453=CARTESIAN_POINT('',(23.5970784790221,3.5,28.6577532024872));
#22454=CARTESIAN_POINT('',(23.5970784790221,2.4,28.6577532024872));
#22455=CARTESIAN_POINT('Origin',(24.2020784790221,3.5,28.6577532024872));
#22456=CARTESIAN_POINT('Origin',(10.5469262078591,2.4,18.4202014332567));
#22457=CARTESIAN_POINT('',(10.3819262078591,2.5,18.4202014332567));
#22458=CARTESIAN_POINT('Origin',(10.5469262078591,2.5,18.4202014332567));
#22459=CARTESIAN_POINT('',(10.3819262078591,3.5,18.4202014332567));
#22460=CARTESIAN_POINT('',(10.3819262078591,2.4,18.4202014332567));
#22461=CARTESIAN_POINT('Origin',(10.5469262078591,3.5,18.4202014332567));
#22462=CARTESIAN_POINT('Origin',(8.82192620785908,2.4,19.4161306476088));
#22463=CARTESIAN_POINT('',(8.65692620785908,2.5,19.4161306476088));
#22464=CARTESIAN_POINT('Origin',(8.82192620785908,2.5,19.4161306476088));
#22465=CARTESIAN_POINT('',(8.65692620785908,3.5,19.4161306476088));
#22466=CARTESIAN_POINT('',(8.65692620785908,2.4,19.4161306476088));
#22467=CARTESIAN_POINT('Origin',(8.82192620785908,3.5,19.4161306476088));
#22468=CARTESIAN_POINT('Origin',(8.82192620785908,2.4,17.4242722189046));
#22469=CARTESIAN_POINT('',(8.65692620785908,2.5,17.4242722189046));
#22470=CARTESIAN_POINT('Origin',(8.82192620785908,2.5,17.4242722189046));
#22471=CARTESIAN_POINT('',(8.65692620785908,3.5,17.4242722189046));
#22472=CARTESIAN_POINT('',(8.65692620785908,2.4,17.4242722189046));
#22473=CARTESIAN_POINT('Origin',(8.82192620785908,3.5,17.4242722189046));
#22474=CARTESIAN_POINT('Origin',(9.39692620785909,2.4,18.4202014332567));
#22475=CARTESIAN_POINT('',(8.79192620785908,2.5,18.4202014332567));
#22476=CARTESIAN_POINT('Origin',(9.39692620785909,2.5,18.4202014332567));
#22477=CARTESIAN_POINT('',(8.79192620785908,3.5,18.4202014332567));
#22478=CARTESIAN_POINT('',(8.79192620785908,2.4,18.4202014332567));
#22479=CARTESIAN_POINT('Origin',(9.39692620785909,3.5,18.4202014332567));
#22480=CARTESIAN_POINT('Origin',(23.0020784790221,2.5,28.6577532024872));
#22481=CARTESIAN_POINT('',(23.0020784790221,2.5,29.9993939889871));
#22482=CARTESIAN_POINT('',(23.0020784790221,3.5,29.9993939889871));
#22483=CARTESIAN_POINT('',(23.0020784790221,2.5,29.9993939889871));
#22484=CARTESIAN_POINT('',(23.0020784790221,2.5,32.));
#22485=CARTESIAN_POINT('',(23.0020784790221,2.5,32.));
#22486=CARTESIAN_POINT('',(23.0020784790221,3.5,32.));
#22487=CARTESIAN_POINT('',(23.0020784790221,2.5,32.));
#22488=CARTESIAN_POINT('',(23.0020784790221,3.5,32.));
#22489=CARTESIAN_POINT('Origin',(25.4020784790221,2.5,32.));
#22490=CARTESIAN_POINT('',(25.4020784790221,3.5,29.9993939889871));
#22491=CARTESIAN_POINT('',(25.4020784790221,2.5,29.9993939889871));
#22492=CARTESIAN_POINT('',(25.4020784790221,2.5,29.9993939889871));
#22493=CARTESIAN_POINT('',(25.4020784790221,3.5,32.));
#22494=CARTESIAN_POINT('',(25.4020784790221,3.5,28.6577532024872));
#22495=CARTESIAN_POINT('',(25.4020784790221,2.5,32.));
#22496=CARTESIAN_POINT('',(25.4020784790221,2.5,32.));
#22497=CARTESIAN_POINT('',(25.4020784790221,2.5,28.6577532024872));
#22498=CARTESIAN_POINT('Origin',(23.0020784790221,2.5,32.));
#22499=CARTESIAN_POINT('',(25.4020784790221,2.5,32.));
#22500=CARTESIAN_POINT('',(25.4020784790221,3.5,32.));
#22501=CARTESIAN_POINT('Origin',(24.2020784790221,2.5,28.6577532024872));
#22502=CARTESIAN_POINT('',(22.4045561490901,3.5,28.7521643956565));
#22503=CARTESIAN_POINT('Origin',(24.2020784790221,3.5,28.6577532024872));
#22504=CARTESIAN_POINT('',(22.4045561490901,2.5,28.7521643956565));
#22505=CARTESIAN_POINT('',(22.4045561490901,2.5,28.7521643956565));
#22506=CARTESIAN_POINT('Origin',(24.2020784790221,2.5,28.6577532024872));
#22507=CARTESIAN_POINT('Origin',(24.2020784790221,2.5,28.6577532024872));
#22508=CARTESIAN_POINT('',(23.6558124764405,2.5,26.9426457847365));
#22509=CARTESIAN_POINT('Origin',(24.2020784790221,2.5,28.6577532024872));
#22510=CARTESIAN_POINT('',(23.6558124764405,3.5,26.9426457847365));
#22511=CARTESIAN_POINT('',(23.6558124764405,2.5,26.9426457847365));
#22512=CARTESIAN_POINT('Origin',(24.2020784790221,3.5,28.6577532024872));
#22513=CARTESIAN_POINT('Origin',(16.7995023434406,2.5,23.538977317872));
#22514=CARTESIAN_POINT('',(10.5969262078591,2.5,20.5873565921787));
#22515=CARTESIAN_POINT('',(8.77129804418388,2.5,19.3249607387167));
#22516=CARTESIAN_POINT('',(10.5969262078591,2.5,32.));
#22517=CARTESIAN_POINT('',(10.5969262078591,2.5,18.4202014332567));
#22518=CARTESIAN_POINT('',(8.19692620785908,2.5,32.));
#22519=CARTESIAN_POINT('',(10.5969262078591,2.5,32.));
#22520=CARTESIAN_POINT('',(8.19692620785908,2.5,19.7618422197566));
#22521=CARTESIAN_POINT('',(8.19692620785908,2.5,32.));
#22522=CARTESIAN_POINT('',(11.1944485377911,2.5,18.3257902400875));
#22523=CARTESIAN_POINT('Origin',(9.39692620785909,2.5,18.4202014332567));
#22524=CARTESIAN_POINT('',(24.8277066426973,2.5,27.7529938970273));
#22525=CARTESIAN_POINT('Origin',(8.19692620785908,2.5,18.4202014332567));
#22526=CARTESIAN_POINT('',(8.19692620785908,3.5,19.7618422197566));
#22527=CARTESIAN_POINT('',(8.19692620785908,2.5,19.7618422197566));
#22528=CARTESIAN_POINT('',(8.19692620785908,3.5,32.));
#22529=CARTESIAN_POINT('',(8.19692620785908,2.5,32.));
#22530=CARTESIAN_POINT('',(8.19692620785908,3.5,32.));
#22531=CARTESIAN_POINT('Origin',(10.5969262078591,2.5,32.));
#22532=CARTESIAN_POINT('',(10.5969262078591,3.5,20.5873565921787));
#22533=CARTESIAN_POINT('',(10.5969262078591,2.5,20.5873565921787));
#22534=CARTESIAN_POINT('',(10.5969262078591,3.5,32.));
#22535=CARTESIAN_POINT('',(10.5969262078591,3.5,18.4202014332567));
#22536=CARTESIAN_POINT('',(10.5969262078591,2.5,32.));
#22537=CARTESIAN_POINT('Origin',(8.19692620785908,2.5,32.));
#22538=CARTESIAN_POINT('',(10.5969262078591,3.5,32.));
#22539=CARTESIAN_POINT('Origin',(8.77129804418388,2.5,19.3249607387167));
#22540=CARTESIAN_POINT('',(8.77129804418388,3.5,19.3249607387167));
#22541=CARTESIAN_POINT('Origin',(9.39692620785909,2.5,18.4202014332567));
#22542=CARTESIAN_POINT('',(11.1944485377911,3.5,18.3257902400875));
#22543=CARTESIAN_POINT('Origin',(9.39692620785909,3.5,18.4202014332567));
#22544=CARTESIAN_POINT('',(11.1944485377911,2.5,18.3257902400875));
#22545=CARTESIAN_POINT('Origin',(24.8277066426973,2.5,27.7529938970273));
#22546=CARTESIAN_POINT('',(24.8277066426973,3.5,27.7529938970273));
#22547=CARTESIAN_POINT('Origin',(16.7995023434406,3.5,23.538977317872));
#22548=CARTESIAN_POINT('Origin',(28.,7.5,32.));
#22549=CARTESIAN_POINT('',(28.,7.5,32.));
#22550=CARTESIAN_POINT('',(8.,7.5,32.));
#22551=CARTESIAN_POINT('',(28.,7.5,32.));
#22552=CARTESIAN_POINT('',(8.,7.5,32.8));
#22553=CARTESIAN_POINT('',(8.,7.5,32.));
#22554=CARTESIAN_POINT('',(28.,7.5,32.8));
#22555=CARTESIAN_POINT('',(28.,7.5,32.8));
#22556=CARTESIAN_POINT('',(28.,7.5,32.));
#22557=CARTESIAN_POINT('Origin',(28.,-3.5,32.));
#22558=CARTESIAN_POINT('',(28.,-3.5,32.));
#22559=CARTESIAN_POINT('',(28.,-3.5,32.));
#22560=CARTESIAN_POINT('',(28.,-3.5,32.8));
#22561=CARTESIAN_POINT('',(28.,-3.5,32.8));
#22562=CARTESIAN_POINT('',(28.,-3.5,32.));
#22563=CARTESIAN_POINT('Origin',(8.,-3.5,32.));
#22564=CARTESIAN_POINT('',(8.,-3.5,32.));
#22565=CARTESIAN_POINT('',(8.,-3.5,32.));
#22566=CARTESIAN_POINT('',(8.,-3.5,32.8));
#22567=CARTESIAN_POINT('',(8.,-3.5,32.8));
#22568=CARTESIAN_POINT('',(8.,-3.5,32.));
#22569=CARTESIAN_POINT('Origin',(8.,7.5,32.));
#22570=CARTESIAN_POINT('',(8.,7.5,32.));
#22571=CARTESIAN_POINT('',(8.,7.5,32.8));
#22572=CARTESIAN_POINT('Origin',(18.,2.,32.8));
#22573=CARTESIAN_POINT('Origin',(18.,2.,32.));
#23578=UNCERTAINTY_MEASURE_WITH_UNIT(LENGTH_MEASURE(0.001),#23729,
'DISTANCE_ACCURACY_VALUE',
'Maximum model space distance between geometric entities at asserted c
onnectivities');
#23611=UNCERTAINTY_MEASURE_WITH_UNIT(LENGTH_MEASURE(0.001),#23729,
'DISTANCE_ACCURACY_VALUE',
'Maximum model space distance between geometric entities at asserted c
onnectivities');
#23695=(
GEOMETRIC_REPRESENTATION_CONTEXT(3)
GLOBAL_UNCERTAINTY_ASSIGNED_CONTEXT((#23578))
GLOBAL_UNIT_ASSIGNED_CONTEXT((#23729,#23731,#23732))
REPRESENTATION_CONTEXT('','3D')
);
#23728=(
GEOMETRIC_REPRESENTATION_CONTEXT(3)
GLOBAL_UNCERTAINTY_ASSIGNED_CONTEXT((#23611))
GLOBAL_UNIT_ASSIGNED_CONTEXT((#23729,#23731,#23732))
REPRESENTATION_CONTEXT('','3D')
);
#23729=(
LENGTH_UNIT()
NAMED_UNIT(*)
SI_UNIT(.CENTI.,.METRE.)
);
#23731=(
NAMED_UNIT(*)
PLANE_ANGLE_UNIT()
SI_UNIT($,.RADIAN.)
);
#23732=(
NAMED_UNIT(*)
SI_UNIT($,.STERADIAN.)
SOLID_ANGLE_UNIT()
);
#23816=SHAPE_DEFINITION_REPRESENTATION(#23983,#24195);
#23983=PRODUCT_DEFINITION_SHAPE('',$,#24312);
#24195=SHAPE_REPRESENTATION('',(#14948),#23695);
#24228=PRODUCT_DEFINITION_CONTEXT('part definition',#24578,'design');
#24312=PRODUCT_DEFINITION('Cradle frame','Cradle frame',#24428,#24228);
#24428=PRODUCT_DEFINITION_FORMATION('',$,#24663);
#24578=APPLICATION_CONTEXT(
'Core Data for Automotive Mechanical Design Process');
#24579=PRODUCT_CONTEXT('part definition',#24578,'mechanical');
#24663=PRODUCT('Cradle frame','Cradle frame','Cradle frame',(#24579));
#24738=COLOUR_RGB('Dark Blue',0.08,0.2,0.34);
#24739=FILL_AREA_STYLE_COLOUR('',#24738);
#24740=FILL_AREA_STYLE('',(#24739));
#24741=SURFACE_STYLE_FILL_AREA(#24740);
#24742=SURFACE_SIDE_STYLE('',(#24741));
#24743=SURFACE_STYLE_USAGE(.BOTH.,#24742);
#24744=PRESENTATION_STYLE_ASSIGNMENT((#24743));
ENDSEC;
END-ISO-10303-21;
